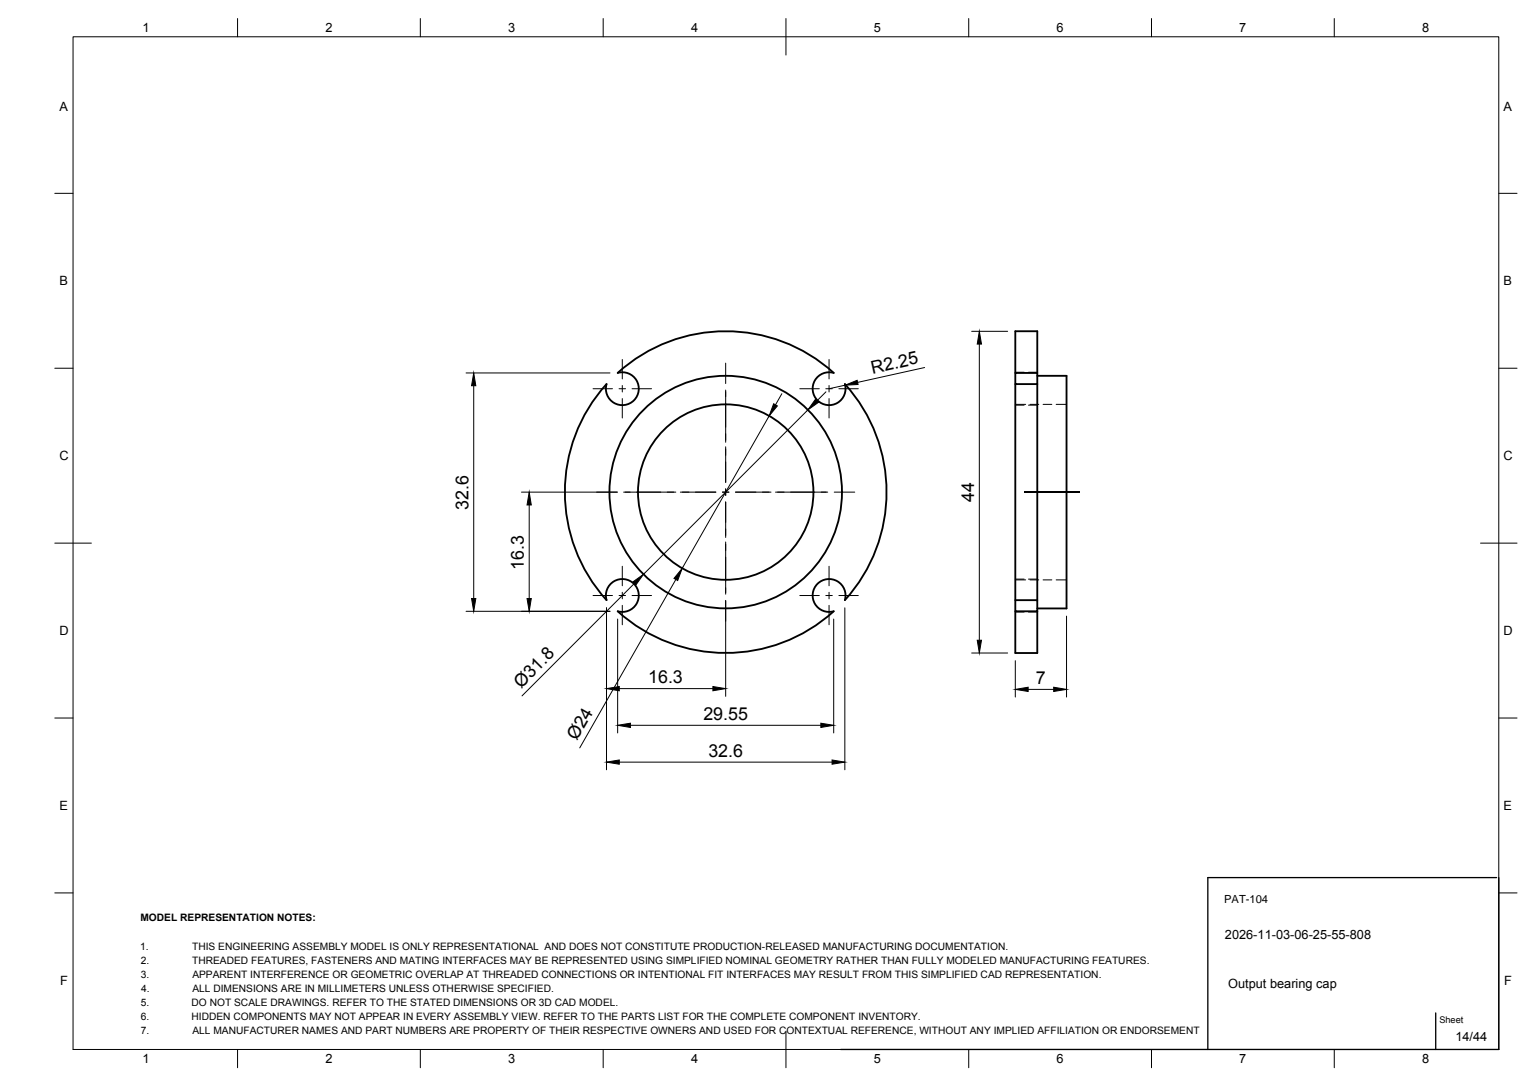
ISO-10303-21;
HEADER;
/* Generated by software containing ST-Developer
 * from STEP Tools, Inc. (www.steptools.com) 
 */

FILE_DESCRIPTION(
/* description */ ('Timing belt drive module 2 mm Pitch Timing 20T-40T'),

/* implementation_level */ '2;1');

FILE_NAME(
/* name */ 'Output bearing cap.step',
/* time_stamp */ '2026-10-28T03:25:12-07:00',
/* author */ (''),
/* organization */ (''),
/* preprocessor_version */ 'ST-DEVELOPER v20.2',
/* originating_system */ 'Autodesk Translation Framework v15.17.0.0',
/* authorisation */ '');

FILE_SCHEMA (('AUTOMOTIVE_DESIGN { 1 0 10303 214 3 1 1 }'));
ENDSEC;

DATA;
#10=MECHANICAL_DESIGN_GEOMETRIC_PRESENTATION_REPRESENTATION('',(#537),#17830);
#451=SHAPE_REPRESENTATION_RELATIONSHIP('SRR','None',#18021,#494);
#494=ADVANCED_BREP_SHAPE_REPRESENTATION('',(#595),#17796);
#537=STYLED_ITEM('',(#18317),#595);
#595=MANIFOLD_SOLID_BREP('Body1',#8994);
#701=FACE_BOUND('',#1682,.T.);
#702=FACE_BOUND('',#1689,.T.);
#703=FACE_BOUND('',#1692,.T.);
#841=PLANE('',#9802);
#842=PLANE('',#9819);
#843=PLANE('',#9822);
#1092=FACE_OUTER_BOUND('',#1677,.T.);
#1093=FACE_OUTER_BOUND('',#1678,.T.);
#1094=FACE_OUTER_BOUND('',#1679,.T.);
#1095=FACE_OUTER_BOUND('',#1680,.T.);
#1096=FACE_OUTER_BOUND('',#1681,.T.);
#1097=FACE_OUTER_BOUND('',#1683,.T.);
#1098=FACE_OUTER_BOUND('',#1684,.T.);
#1099=FACE_OUTER_BOUND('',#1685,.T.);
#1100=FACE_OUTER_BOUND('',#1686,.T.);
#1101=FACE_OUTER_BOUND('',#1687,.T.);
#1102=FACE_OUTER_BOUND('',#1688,.T.);
#1103=FACE_OUTER_BOUND('',#1690,.T.);
#1104=FACE_OUTER_BOUND('',#1691,.T.);
#1677=EDGE_LOOP('',(#6373,#6374,#6375,#6376));
#1678=EDGE_LOOP('',(#6377,#6378,#6379,#6380));
#1679=EDGE_LOOP('',(#6381,#6382,#6383,#6384));
#1680=EDGE_LOOP('',(#6385,#6386,#6387,#6388));
#1681=EDGE_LOOP('',(#6389,#6390,#6391,#6392,#6393,#6394,#6395,#6396));
#1682=EDGE_LOOP('',(#6397));
#1683=EDGE_LOOP('',(#6398,#6399,#6400,#6401));
#1684=EDGE_LOOP('',(#6402,#6403,#6404,#6405));
#1685=EDGE_LOOP('',(#6406,#6407,#6408,#6409));
#1686=EDGE_LOOP('',(#6410,#6411,#6412,#6413));
#1687=EDGE_LOOP('',(#6414,#6415,#6416,#6417));
#1688=EDGE_LOOP('',(#6418));
#1689=EDGE_LOOP('',(#6419));
#1690=EDGE_LOOP('',(#6420,#6421,#6422,#6423));
#1691=EDGE_LOOP('',(#6424,#6425,#6426,#6427,#6428,#6429,#6430,#6431));
#1692=EDGE_LOOP('',(#6432));
#2268=CIRCLE('',#9791,0.225);
#2269=CIRCLE('',#9792,0.225);
#2270=CIRCLE('',#9794,0.225);
#2271=CIRCLE('',#9795,0.225);
#2272=CIRCLE('',#9797,0.225);
#2273=CIRCLE('',#9798,0.225);
#2274=CIRCLE('',#9800,0.225);
#2275=CIRCLE('',#9801,0.225);
#2276=CIRCLE('',#9803,2.2);
#2277=CIRCLE('',#9804,2.2);
#2278=CIRCLE('',#9805,2.2);
#2279=CIRCLE('',#9806,2.2);
#2280=CIRCLE('',#9807,1.2);
#2281=CIRCLE('',#9809,2.2);
#2282=CIRCLE('',#9811,2.2);
#2283=CIRCLE('',#9813,2.2);
#2284=CIRCLE('',#9815,2.2);
#2285=CIRCLE('',#9817,1.59);
#2286=CIRCLE('',#9818,1.59);
#2287=CIRCLE('',#9820,1.2);
#2962=LINE('',#14522,#3440);
#2963=LINE('',#14526,#3441);
#2964=LINE('',#14531,#3442);
#2965=LINE('',#14535,#3443);
#2966=LINE('',#14540,#3444);
#2967=LINE('',#14544,#3445);
#2968=LINE('',#14549,#3446);
#2969=LINE('',#14553,#3447);
#2970=LINE('',#14574,#3448);
#2971=LINE('',#14580,#3449);
#3440=VECTOR('',#11531,1.);
#3441=VECTOR('',#11534,1.);
#3442=VECTOR('',#11539,1.);
#3443=VECTOR('',#11542,1.);
#3444=VECTOR('',#11547,1.);
#3445=VECTOR('',#11550,1.);
#3446=VECTOR('',#11555,1.);
#3447=VECTOR('',#11558,1.);
#3448=VECTOR('',#11593,1.59);
#3449=VECTOR('',#11602,1.2);
#3946=VERTEX_POINT('',#14520);
#3947=VERTEX_POINT('',#14521);
#3948=VERTEX_POINT('',#14523);
#3949=VERTEX_POINT('',#14525);
#3950=VERTEX_POINT('',#14529);
#3951=VERTEX_POINT('',#14530);
#3952=VERTEX_POINT('',#14532);
#3953=VERTEX_POINT('',#14534);
#3954=VERTEX_POINT('',#14538);
#3955=VERTEX_POINT('',#14539);
#3956=VERTEX_POINT('',#14541);
#3957=VERTEX_POINT('',#14543);
#3958=VERTEX_POINT('',#14547);
#3959=VERTEX_POINT('',#14548);
#3960=VERTEX_POINT('',#14550);
#3961=VERTEX_POINT('',#14552);
#3962=VERTEX_POINT('',#14560);
#3963=VERTEX_POINT('',#14571);
#3964=VERTEX_POINT('',#14573);
#3965=VERTEX_POINT('',#14577);
#4869=EDGE_CURVE('',#3946,#3947,#2962,.T.);
#4870=EDGE_CURVE('',#3948,#3946,#2268,.T.);
#4871=EDGE_CURVE('',#3949,#3948,#2963,.T.);
#4872=EDGE_CURVE('',#3947,#3949,#2269,.T.);
#4873=EDGE_CURVE('',#3950,#3951,#2964,.T.);
#4874=EDGE_CURVE('',#3952,#3950,#2270,.T.);
#4875=EDGE_CURVE('',#3953,#3952,#2965,.T.);
#4876=EDGE_CURVE('',#3951,#3953,#2271,.T.);
#4877=EDGE_CURVE('',#3954,#3955,#2966,.T.);
#4878=EDGE_CURVE('',#3956,#3954,#2272,.T.);
#4879=EDGE_CURVE('',#3957,#3956,#2967,.T.);
#4880=EDGE_CURVE('',#3955,#3957,#2273,.T.);
#4881=EDGE_CURVE('',#3958,#3959,#2968,.T.);
#4882=EDGE_CURVE('',#3960,#3958,#2274,.T.);
#4883=EDGE_CURVE('',#3961,#3960,#2969,.T.);
#4884=EDGE_CURVE('',#3959,#3961,#2275,.T.);
#4885=EDGE_CURVE('',#3960,#3946,#2276,.T.);
#4886=EDGE_CURVE('',#3956,#3958,#2277,.T.);
#4887=EDGE_CURVE('',#3952,#3954,#2278,.T.);
#4888=EDGE_CURVE('',#3948,#3950,#2279,.T.);
#4889=EDGE_CURVE('',#3962,#3962,#2280,.T.);
#4890=EDGE_CURVE('',#3957,#3959,#2281,.T.);
#4891=EDGE_CURVE('',#3953,#3955,#2282,.T.);
#4892=EDGE_CURVE('',#3961,#3947,#2283,.T.);
#4893=EDGE_CURVE('',#3949,#3951,#2284,.T.);
#4894=EDGE_CURVE('',#3963,#3963,#2285,.T.);
#4895=EDGE_CURVE('',#3963,#3964,#2970,.T.);
#4896=EDGE_CURVE('',#3964,#3964,#2286,.T.);
#4897=EDGE_CURVE('',#3965,#3965,#2287,.T.);
#4898=EDGE_CURVE('',#3965,#3962,#2971,.T.);
#6373=ORIENTED_EDGE('',*,*,#4869,.F.);
#6374=ORIENTED_EDGE('',*,*,#4870,.F.);
#6375=ORIENTED_EDGE('',*,*,#4871,.F.);
#6376=ORIENTED_EDGE('',*,*,#4872,.F.);
#6377=ORIENTED_EDGE('',*,*,#4873,.F.);
#6378=ORIENTED_EDGE('',*,*,#4874,.F.);
#6379=ORIENTED_EDGE('',*,*,#4875,.F.);
#6380=ORIENTED_EDGE('',*,*,#4876,.F.);
#6381=ORIENTED_EDGE('',*,*,#4877,.F.);
#6382=ORIENTED_EDGE('',*,*,#4878,.F.);
#6383=ORIENTED_EDGE('',*,*,#4879,.F.);
#6384=ORIENTED_EDGE('',*,*,#4880,.F.);
#6385=ORIENTED_EDGE('',*,*,#4881,.F.);
#6386=ORIENTED_EDGE('',*,*,#4882,.F.);
#6387=ORIENTED_EDGE('',*,*,#4883,.F.);
#6388=ORIENTED_EDGE('',*,*,#4884,.F.);
#6389=ORIENTED_EDGE('',*,*,#4870,.T.);
#6390=ORIENTED_EDGE('',*,*,#4885,.F.);
#6391=ORIENTED_EDGE('',*,*,#4882,.T.);
#6392=ORIENTED_EDGE('',*,*,#4886,.F.);
#6393=ORIENTED_EDGE('',*,*,#4878,.T.);
#6394=ORIENTED_EDGE('',*,*,#4887,.F.);
#6395=ORIENTED_EDGE('',*,*,#4874,.T.);
#6396=ORIENTED_EDGE('',*,*,#4888,.F.);
#6397=ORIENTED_EDGE('',*,*,#4889,.F.);
#6398=ORIENTED_EDGE('',*,*,#4879,.T.);
#6399=ORIENTED_EDGE('',*,*,#4886,.T.);
#6400=ORIENTED_EDGE('',*,*,#4881,.T.);
#6401=ORIENTED_EDGE('',*,*,#4890,.F.);
#6402=ORIENTED_EDGE('',*,*,#4875,.T.);
#6403=ORIENTED_EDGE('',*,*,#4887,.T.);
#6404=ORIENTED_EDGE('',*,*,#4877,.T.);
#6405=ORIENTED_EDGE('',*,*,#4891,.F.);
#6406=ORIENTED_EDGE('',*,*,#4869,.T.);
#6407=ORIENTED_EDGE('',*,*,#4892,.F.);
#6408=ORIENTED_EDGE('',*,*,#4883,.T.);
#6409=ORIENTED_EDGE('',*,*,#4885,.T.);
#6410=ORIENTED_EDGE('',*,*,#4871,.T.);
#6411=ORIENTED_EDGE('',*,*,#4888,.T.);
#6412=ORIENTED_EDGE('',*,*,#4873,.T.);
#6413=ORIENTED_EDGE('',*,*,#4893,.F.);
#6414=ORIENTED_EDGE('',*,*,#4894,.F.);
#6415=ORIENTED_EDGE('',*,*,#4895,.T.);
#6416=ORIENTED_EDGE('',*,*,#4896,.F.);
#6417=ORIENTED_EDGE('',*,*,#4895,.F.);
#6418=ORIENTED_EDGE('',*,*,#4894,.T.);
#6419=ORIENTED_EDGE('',*,*,#4897,.T.);
#6420=ORIENTED_EDGE('',*,*,#4897,.F.);
#6421=ORIENTED_EDGE('',*,*,#4898,.T.);
#6422=ORIENTED_EDGE('',*,*,#4889,.T.);
#6423=ORIENTED_EDGE('',*,*,#4898,.F.);
#6424=ORIENTED_EDGE('',*,*,#4872,.T.);
#6425=ORIENTED_EDGE('',*,*,#4893,.T.);
#6426=ORIENTED_EDGE('',*,*,#4876,.T.);
#6427=ORIENTED_EDGE('',*,*,#4891,.T.);
#6428=ORIENTED_EDGE('',*,*,#4880,.T.);
#6429=ORIENTED_EDGE('',*,*,#4890,.T.);
#6430=ORIENTED_EDGE('',*,*,#4884,.T.);
#6431=ORIENTED_EDGE('',*,*,#4892,.T.);
#6432=ORIENTED_EDGE('',*,*,#4896,.T.);
#8243=CYLINDRICAL_SURFACE('',#9790,0.225);
#8244=CYLINDRICAL_SURFACE('',#9793,0.225);
#8245=CYLINDRICAL_SURFACE('',#9796,0.225);
#8246=CYLINDRICAL_SURFACE('',#9799,0.225);
#8247=CYLINDRICAL_SURFACE('',#9808,2.2);
#8248=CYLINDRICAL_SURFACE('',#9810,2.2);
#8249=CYLINDRICAL_SURFACE('',#9812,2.2);
#8250=CYLINDRICAL_SURFACE('',#9814,2.2);
#8251=CYLINDRICAL_SURFACE('',#9816,1.59);
#8252=CYLINDRICAL_SURFACE('',#9821,1.2);
#8590=ADVANCED_FACE('',(#1092),#8243,.F.);
#8591=ADVANCED_FACE('',(#1093),#8244,.F.);
#8592=ADVANCED_FACE('',(#1094),#8245,.F.);
#8593=ADVANCED_FACE('',(#1095),#8246,.F.);
#8594=ADVANCED_FACE('',(#1096,#701),#841,.F.);
#8595=ADVANCED_FACE('',(#1097),#8247,.T.);
#8596=ADVANCED_FACE('',(#1098),#8248,.T.);
#8597=ADVANCED_FACE('',(#1099),#8249,.T.);
#8598=ADVANCED_FACE('',(#1100),#8250,.T.);
#8599=ADVANCED_FACE('',(#1101),#8251,.T.);
#8600=ADVANCED_FACE('',(#1102,#702),#842,.T.);
#8601=ADVANCED_FACE('',(#1103),#8252,.F.);
#8602=ADVANCED_FACE('',(#1104,#703),#843,.T.);
#8994=CLOSED_SHELL('',(#8590,#8591,#8592,#8593,#8594,#8595,#8596,#8597,
#8598,#8599,#8600,#8601,#8602));
#9789=AXIS2_PLACEMENT_3D('',#14518,#11527,#11528);
#9790=AXIS2_PLACEMENT_3D('',#14519,#11529,#11530);
#9791=AXIS2_PLACEMENT_3D('',#14524,#11532,#11533);
#9792=AXIS2_PLACEMENT_3D('',#14527,#11535,#11536);
#9793=AXIS2_PLACEMENT_3D('',#14528,#11537,#11538);
#9794=AXIS2_PLACEMENT_3D('',#14533,#11540,#11541);
#9795=AXIS2_PLACEMENT_3D('',#14536,#11543,#11544);
#9796=AXIS2_PLACEMENT_3D('',#14537,#11545,#11546);
#9797=AXIS2_PLACEMENT_3D('',#14542,#11548,#11549);
#9798=AXIS2_PLACEMENT_3D('',#14545,#11551,#11552);
#9799=AXIS2_PLACEMENT_3D('',#14546,#11553,#11554);
#9800=AXIS2_PLACEMENT_3D('',#14551,#11556,#11557);
#9801=AXIS2_PLACEMENT_3D('',#14554,#11559,#11560);
#9802=AXIS2_PLACEMENT_3D('',#14555,#11561,#11562);
#9803=AXIS2_PLACEMENT_3D('',#14556,#11563,#11564);
#9804=AXIS2_PLACEMENT_3D('',#14557,#11565,#11566);
#9805=AXIS2_PLACEMENT_3D('',#14558,#11567,#11568);
#9806=AXIS2_PLACEMENT_3D('',#14559,#11569,#11570);
#9807=AXIS2_PLACEMENT_3D('',#14561,#11571,#11572);
#9808=AXIS2_PLACEMENT_3D('',#14562,#11573,#11574);
#9809=AXIS2_PLACEMENT_3D('',#14563,#11575,#11576);
#9810=AXIS2_PLACEMENT_3D('',#14564,#11577,#11578);
#9811=AXIS2_PLACEMENT_3D('',#14565,#11579,#11580);
#9812=AXIS2_PLACEMENT_3D('',#14566,#11581,#11582);
#9813=AXIS2_PLACEMENT_3D('',#14567,#11583,#11584);
#9814=AXIS2_PLACEMENT_3D('',#14568,#11585,#11586);
#9815=AXIS2_PLACEMENT_3D('',#14569,#11587,#11588);
#9816=AXIS2_PLACEMENT_3D('',#14570,#11589,#11590);
#9817=AXIS2_PLACEMENT_3D('',#14572,#11591,#11592);
#9818=AXIS2_PLACEMENT_3D('',#14575,#11594,#11595);
#9819=AXIS2_PLACEMENT_3D('',#14576,#11596,#11597);
#9820=AXIS2_PLACEMENT_3D('',#14578,#11598,#11599);
#9821=AXIS2_PLACEMENT_3D('',#14579,#11600,#11601);
#9822=AXIS2_PLACEMENT_3D('',#14581,#11603,#11604);
#11527=DIRECTION('axis',(0.,0.,1.));
#11528=DIRECTION('refdir',(1.,0.,0.));
#11529=DIRECTION('center_axis',(0.,1.,0.));
#11530=DIRECTION('ref_axis',(0.707106781186546,0.,0.707106781186549));
#11531=DIRECTION('',(0.,1.,0.));
#11532=DIRECTION('center_axis',(0.,1.,0.));
#11533=DIRECTION('ref_axis',(1.,0.,0.));
#11534=DIRECTION('',(0.,-1.,0.));
#11535=DIRECTION('center_axis',(0.,-1.,0.));
#11536=DIRECTION('ref_axis',(1.,0.,0.));
#11537=DIRECTION('center_axis',(0.,1.,0.));
#11538=DIRECTION('ref_axis',(0.707106781186544,0.,-0.707106781186551));
#11539=DIRECTION('',(0.,1.,0.));
#11540=DIRECTION('center_axis',(0.,1.,0.));
#11541=DIRECTION('ref_axis',(1.,0.,0.));
#11542=DIRECTION('',(0.,-1.,0.));
#11543=DIRECTION('center_axis',(0.,-1.,0.));
#11544=DIRECTION('ref_axis',(1.,0.,0.));
#11545=DIRECTION('center_axis',(0.,1.,0.));
#11546=DIRECTION('ref_axis',(-0.707106781186548,0.,-0.707106781186547));
#11547=DIRECTION('',(0.,1.,0.));
#11548=DIRECTION('center_axis',(0.,1.,0.));
#11549=DIRECTION('ref_axis',(1.,0.,0.));
#11550=DIRECTION('',(0.,-1.,0.));
#11551=DIRECTION('center_axis',(0.,-1.,0.));
#11552=DIRECTION('ref_axis',(1.,0.,0.));
#11553=DIRECTION('center_axis',(0.,1.,0.));
#11554=DIRECTION('ref_axis',(-0.707106781186544,0.,0.707106781186551));
#11555=DIRECTION('',(0.,1.,0.));
#11556=DIRECTION('center_axis',(0.,1.,0.));
#11557=DIRECTION('ref_axis',(1.,0.,0.));
#11558=DIRECTION('',(0.,-1.,0.));
#11559=DIRECTION('center_axis',(0.,-1.,0.));
#11560=DIRECTION('ref_axis',(1.,0.,0.));
#11561=DIRECTION('center_axis',(0.,1.,0.));
#11562=DIRECTION('ref_axis',(1.,0.,0.));
#11563=DIRECTION('center_axis',(0.,1.,0.));
#11564=DIRECTION('ref_axis',(1.,0.,0.));
#11565=DIRECTION('center_axis',(0.,1.,0.));
#11566=DIRECTION('ref_axis',(1.,0.,0.));
#11567=DIRECTION('center_axis',(0.,1.,0.));
#11568=DIRECTION('ref_axis',(1.,0.,0.));
#11569=DIRECTION('center_axis',(0.,1.,0.));
#11570=DIRECTION('ref_axis',(1.,0.,0.));
#11571=DIRECTION('center_axis',(0.,-1.,0.));
#11572=DIRECTION('ref_axis',(1.,0.,0.));
#11573=DIRECTION('center_axis',(0.,1.,0.));
#11574=DIRECTION('ref_axis',(1.,0.,0.));
#11575=DIRECTION('center_axis',(0.,1.,0.));
#11576=DIRECTION('ref_axis',(1.,0.,0.));
#11577=DIRECTION('center_axis',(0.,1.,0.));
#11578=DIRECTION('ref_axis',(1.,0.,0.));
#11579=DIRECTION('center_axis',(0.,1.,0.));
#11580=DIRECTION('ref_axis',(1.,0.,0.));
#11581=DIRECTION('center_axis',(0.,1.,0.));
#11582=DIRECTION('ref_axis',(1.,0.,0.));
#11583=DIRECTION('center_axis',(0.,1.,0.));
#11584=DIRECTION('ref_axis',(1.,0.,0.));
#11585=DIRECTION('center_axis',(0.,1.,0.));
#11586=DIRECTION('ref_axis',(-1.,0.,-1.01064309961486E-15));
#11587=DIRECTION('center_axis',(0.,1.,0.));
#11588=DIRECTION('ref_axis',(1.,0.,0.));
#11589=DIRECTION('center_axis',(0.,1.,0.));
#11590=DIRECTION('ref_axis',(1.,0.,0.));
#11591=DIRECTION('center_axis',(0.,1.,0.));
#11592=DIRECTION('ref_axis',(1.,0.,0.));
#11593=DIRECTION('',(0.,-1.,0.));
#11594=DIRECTION('center_axis',(0.,-1.,0.));
#11595=DIRECTION('ref_axis',(1.,0.,0.));
#11596=DIRECTION('center_axis',(0.,1.,0.));
#11597=DIRECTION('ref_axis',(1.,0.,0.));
#11598=DIRECTION('center_axis',(0.,-1.,0.));
#11599=DIRECTION('ref_axis',(1.,0.,0.));
#11600=DIRECTION('center_axis',(0.,1.,0.));
#11601=DIRECTION('ref_axis',(1.,0.,0.));
#11602=DIRECTION('',(0.,-1.,0.));
#11603=DIRECTION('center_axis',(0.,1.,0.));
#11604=DIRECTION('ref_axis',(1.,0.,0.));
#14518=CARTESIAN_POINT('',(0.,0.,0.));
#14519=CARTESIAN_POINT('Origin',(5.55669646780806,-2.2,5.58578643762691));
#14520=CARTESIAN_POINT('',(5.49357471024299,-2.1,5.36982198749241));
#14521=CARTESIAN_POINT('',(5.49357471024299,-1.8,5.36982198749241));
#14522=CARTESIAN_POINT('',(5.49357471024299,-2.2,5.36982198749241));
#14523=CARTESIAN_POINT('',(5.34073201767356,-2.1,5.52266468006184));
#14524=CARTESIAN_POINT('Origin',(5.55669646780806,-2.1,5.58578643762691));
#14525=CARTESIAN_POINT('',(5.34073201767356,-1.8,5.52266468006184));
#14526=CARTESIAN_POINT('',(5.34073201767356,-2.2,5.52266468006184));
#14527=CARTESIAN_POINT('Origin',(5.55669646780806,-1.8,5.58578643762691));
#14528=CARTESIAN_POINT('Origin',(5.55669646780806,-2.2,8.4142135623731));
#14529=CARTESIAN_POINT('',(5.34073201767356,-2.1,8.47733531993816));
#14530=CARTESIAN_POINT('',(5.34073201767356,-1.8,8.47733531993816));
#14531=CARTESIAN_POINT('',(5.34073201767356,-2.2,8.47733531993816));
#14532=CARTESIAN_POINT('',(5.493574710243,-2.1,8.6301780125076));
#14533=CARTESIAN_POINT('Origin',(5.55669646780806,-2.1,8.4142135623731));
#14534=CARTESIAN_POINT('',(5.493574710243,-1.8,8.6301780125076));
#14535=CARTESIAN_POINT('',(5.493574710243,-2.2,8.6301780125076));
#14536=CARTESIAN_POINT('Origin',(5.55669646780806,-1.8,8.4142135623731));
#14537=CARTESIAN_POINT('Origin',(8.38512359255425,-2.2,8.4142135623731));
#14538=CARTESIAN_POINT('',(8.44824535011931,-2.1,8.6301780125076));
#14539=CARTESIAN_POINT('',(8.44824535011931,-1.8,8.6301780125076));
#14540=CARTESIAN_POINT('',(8.44824535011932,-2.2,8.6301780125076));
#14541=CARTESIAN_POINT('',(8.60108804268875,-2.1,8.47733531993816));
#14542=CARTESIAN_POINT('Origin',(8.38512359255425,-2.1,8.4142135623731));
#14543=CARTESIAN_POINT('',(8.60108804268875,-1.8,8.47733531993816));
#14544=CARTESIAN_POINT('',(8.60108804268875,-2.2,8.47733531993816));
#14545=CARTESIAN_POINT('Origin',(8.38512359255425,-1.8,8.4142135623731));
#14546=CARTESIAN_POINT('Origin',(8.38512359255425,-2.2,5.58578643762691));
#14547=CARTESIAN_POINT('',(8.60108804268875,-2.1,5.52266468006184));
#14548=CARTESIAN_POINT('',(8.60108804268875,-1.8,5.52266468006184));
#14549=CARTESIAN_POINT('',(8.60108804268875,-2.2,5.52266468006184));
#14550=CARTESIAN_POINT('',(8.44824535011932,-2.1,5.36982198749241));
#14551=CARTESIAN_POINT('Origin',(8.38512359255425,-2.1,5.58578643762691));
#14552=CARTESIAN_POINT('',(8.44824535011932,-1.8,5.36982198749241));
#14553=CARTESIAN_POINT('',(8.44824535011932,-2.2,5.36982198749241));
#14554=CARTESIAN_POINT('Origin',(8.38512359255425,-1.8,5.58578643762691));
#14555=CARTESIAN_POINT('Origin',(6.97091003018116,-2.1,7.));
#14556=CARTESIAN_POINT('Origin',(6.97091003018116,-2.1,7.));
#14557=CARTESIAN_POINT('Origin',(6.97091003018116,-2.1,7.));
#14558=CARTESIAN_POINT('Origin',(6.97091003018116,-2.1,7.));
#14559=CARTESIAN_POINT('Origin',(6.97091003018116,-2.1,7.));
#14560=CARTESIAN_POINT('',(5.77091003018116,-2.1,7.));
#14561=CARTESIAN_POINT('Origin',(6.97091003018116,-2.1,7.));
#14562=CARTESIAN_POINT('Origin',(6.97091003018116,-2.1,7.));
#14563=CARTESIAN_POINT('Origin',(6.97091003018116,-1.8,7.));
#14564=CARTESIAN_POINT('Origin',(6.97091003018116,-2.1,7.));
#14565=CARTESIAN_POINT('Origin',(6.97091003018116,-1.8,7.));
#14566=CARTESIAN_POINT('Origin',(6.97091003018116,-2.1,7.));
#14567=CARTESIAN_POINT('Origin',(6.97091003018116,-1.8,7.));
#14568=CARTESIAN_POINT('Origin',(6.97091003018116,-2.1,7.));
#14569=CARTESIAN_POINT('Origin',(6.97091003018116,-1.8,7.));
#14570=CARTESIAN_POINT('Origin',(6.97091003018116,-1.8,7.));
#14571=CARTESIAN_POINT('',(5.38091003018116,-1.4,7.));
#14572=CARTESIAN_POINT('Origin',(6.97091003018116,-1.4,7.));
#14573=CARTESIAN_POINT('',(5.38091003018116,-1.8,7.));
#14574=CARTESIAN_POINT('',(5.38091003018116,-1.8,7.));
#14575=CARTESIAN_POINT('Origin',(6.97091003018116,-1.8,7.));
#14576=CARTESIAN_POINT('Origin',(6.97091003018116,-1.4,7.));
#14577=CARTESIAN_POINT('',(5.77091003018116,-1.4,7.));
#14578=CARTESIAN_POINT('Origin',(6.97091003018116,-1.4,7.));
#14579=CARTESIAN_POINT('Origin',(6.97091003018116,-2.1,7.));
#14580=CARTESIAN_POINT('',(5.77091003018116,-2.1,7.));
#14581=CARTESIAN_POINT('Origin',(6.97091003018116,-1.8,7.));
#17746=UNCERTAINTY_MEASURE_WITH_UNIT(LENGTH_MEASURE(0.001),#17831,
'DISTANCE_ACCURACY_VALUE',
'Maximum model space distance between geometric entities at asserted c
onnectivities');
#17780=UNCERTAINTY_MEASURE_WITH_UNIT(LENGTH_MEASURE(0.001),#17831,
'DISTANCE_ACCURACY_VALUE',
'Maximum model space distance between geometric entities at asserted c
onnectivities');
#17796=(
GEOMETRIC_REPRESENTATION_CONTEXT(3)
GLOBAL_UNCERTAINTY_ASSIGNED_CONTEXT((#17746))
GLOBAL_UNIT_ASSIGNED_CONTEXT((#17831,#17833,#17834))
REPRESENTATION_CONTEXT('','3D')
);
#17830=(
GEOMETRIC_REPRESENTATION_CONTEXT(3)
GLOBAL_UNCERTAINTY_ASSIGNED_CONTEXT((#17780))
GLOBAL_UNIT_ASSIGNED_CONTEXT((#17831,#17833,#17834))
REPRESENTATION_CONTEXT('','3D')
);
#17831=(
LENGTH_UNIT()
NAMED_UNIT(*)
SI_UNIT(.CENTI.,.METRE.)
);
#17833=(
NAMED_UNIT(*)
PLANE_ANGLE_UNIT()
SI_UNIT($,.RADIAN.)
);
#17834=(
NAMED_UNIT(*)
SI_UNIT($,.STERADIAN.)
SOLID_ANGLE_UNIT()
);
#17850=SHAPE_DEFINITION_REPRESENTATION(#17899,#18021);
#17899=PRODUCT_DEFINITION_SHAPE('',$,#18071);
#18021=SHAPE_REPRESENTATION('',(#9789),#17796);
#18055=PRODUCT_DEFINITION_CONTEXT('part definition',#18204,'design');
#18071=PRODUCT_DEFINITION('Output bearing cap','Output bearing cap',#18120,
#18055);
#18120=PRODUCT_DEFINITION_FORMATION('',$,#18221);
#18204=APPLICATION_CONTEXT(
'Core Data for Automotive Mechanical Design Process');
#18205=PRODUCT_CONTEXT('part definition',#18204,'mechanical');
#18221=PRODUCT('Output bearing cap','Output bearing cap',
'Output bearing cap',(#18205));
#18311=COLOUR_RGB('Grey',0.48,0.52,0.57);
#18312=FILL_AREA_STYLE_COLOUR('',#18311);
#18313=FILL_AREA_STYLE('',(#18312));
#18314=SURFACE_STYLE_FILL_AREA(#18313);
#18315=SURFACE_SIDE_STYLE('',(#18314));
#18316=SURFACE_STYLE_USAGE(.BOTH.,#18315);
#18317=PRESENTATION_STYLE_ASSIGNMENT((#18316));
ENDSEC;
END-ISO-10303-21;
